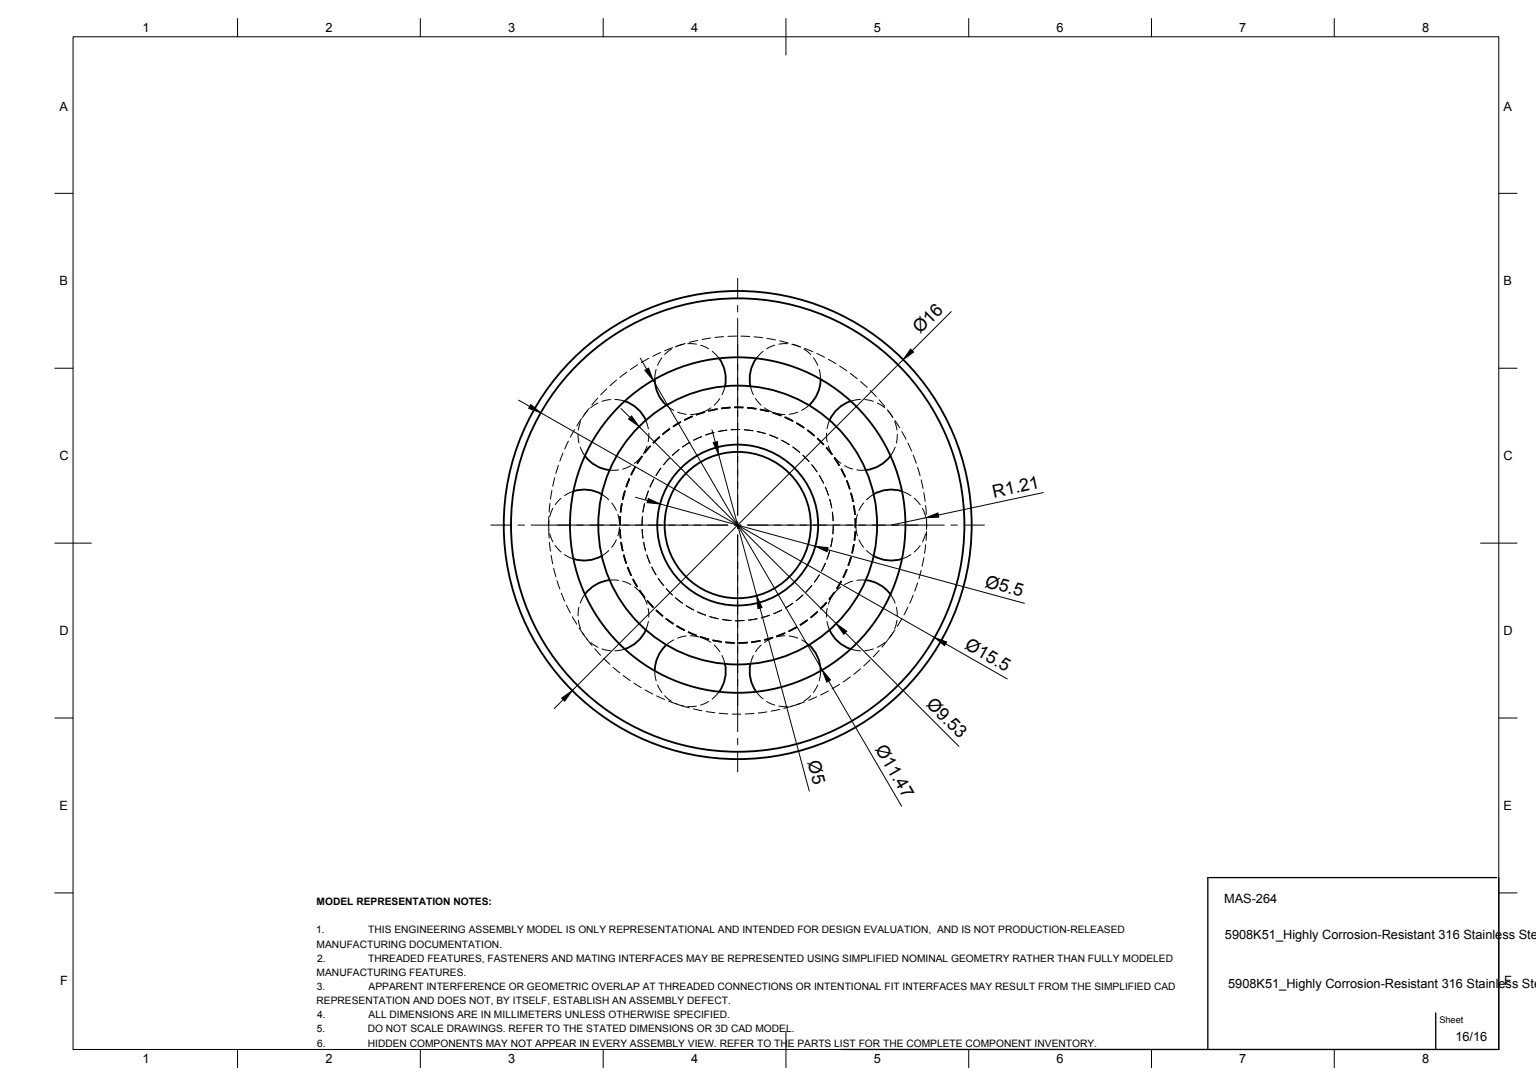
ISO-10303-21;
HEADER;
/* Generated by software containing ST-Developer
 * from STEP Tools, Inc. (www.steptools.com) 
 */

FILE_DESCRIPTION(
/* description */ (''),
/* implementation_level */ '2;1');

FILE_NAME(
/* name */ '5908K51_Highly Corrosion-Resistant 316 Stainless Steel Ball Bearing.step',
/* time_stamp */ '2026-10-12T15:37:13-07:00',
/* author */ (''),
/* organization */ (''),
/* preprocessor_version */ 'ST-DEVELOPER v20.2',
/* originating_system */ 'Autodesk Translation Framework v15.15.0.0',
/* authorisation */ '');

FILE_SCHEMA (('AUTOMOTIVE_DESIGN { 1 0 10303 214 3 1 1 }'));
ENDSEC;

DATA;
#10=MECHANICAL_DESIGN_GEOMETRIC_PRESENTATION_REPRESENTATION('',(#337,#338,#339,#340,#341,#342,#343,#344,#345,#346,#347,#348,#349),#36460);
#95=SPHERICAL_SURFACE('',#11984,1.21175743903915);
#96=SPHERICAL_SURFACE('',#11986,1.21175743903915);
#97=SPHERICAL_SURFACE('',#11988,1.21175743903915);
#98=SPHERICAL_SURFACE('',#11990,1.21175743903915);
#99=SPHERICAL_SURFACE('',#11992,1.21175743903915);
#100=SPHERICAL_SURFACE('',#11994,1.21175743903915);
#101=SPHERICAL_SURFACE('',#11996,1.21175743903915);
#102=SPHERICAL_SURFACE('',#11998,1.21175743903915);
#103=SPHERICAL_SURFACE('',#12000,1.21175743903915);
#104=SPHERICAL_SURFACE('',#12002,1.21175743903915);
#110=SHAPE_REPRESENTATION_RELATIONSHIP('SRR','None',#36522,#123);
#123=ADVANCED_BREP_SHAPE_REPRESENTATION('',(#369,#370,#371,#372,#373,#374,
#375,#376,#377,#378,#379,#380,#381),#36451);
#165=FACE_BOUND('',#2009,.T.);
#166=FACE_BOUND('',#2011,.T.);
#167=FACE_BOUND('',#2017,.T.);
#168=FACE_BOUND('',#2019,.T.);
#169=FACE_BOUND('',#2028,.T.);
#170=FACE_BOUND('',#2030,.T.);
#171=FACE_BOUND('',#2032,.T.);
#319=CONICAL_SURFACE('',#11939,7.75,0.785398163397447);
#320=CONICAL_SURFACE('',#11945,8.,0.785398163397448);
#321=CONICAL_SURFACE('',#11958,4.01780239848197,0.78539816339745);
#322=CONICAL_SURFACE('',#11962,3.26912128048043,0.78539816339745);
#323=CONICAL_SURFACE('',#11968,2.5,0.785398163397447);
#324=CONICAL_SURFACE('',#11979,3.26912128048043,0.78539816339745);
#337=STYLED_ITEM('',(#36596),#369);
#338=STYLED_ITEM('',(#36596),#370);
#339=STYLED_ITEM('',(#36596),#371);
#340=STYLED_ITEM('',(#36596),#372);
#341=STYLED_ITEM('',(#36596),#373);
#342=STYLED_ITEM('',(#36596),#374);
#343=STYLED_ITEM('',(#36596),#375);
#344=STYLED_ITEM('',(#36596),#376);
#345=STYLED_ITEM('',(#36596),#377);
#346=STYLED_ITEM('',(#36596),#378);
#347=STYLED_ITEM('',(#36596),#379);
#348=STYLED_ITEM('',(#36596),#380);
#349=STYLED_ITEM('',(#36596),#381);
#369=MANIFOLD_SOLID_BREP('Body1',#11273);
#370=MANIFOLD_SOLID_BREP('Body2',#11274);
#371=MANIFOLD_SOLID_BREP('Body3',#11275);
#372=MANIFOLD_SOLID_BREP('Body4',#11276);
#373=MANIFOLD_SOLID_BREP('Body5',#11277);
#374=MANIFOLD_SOLID_BREP('Body6',#11278);
#375=MANIFOLD_SOLID_BREP('Body7',#11279);
#376=MANIFOLD_SOLID_BREP('Body8',#11280);
#377=MANIFOLD_SOLID_BREP('Body9',#11281);
#378=MANIFOLD_SOLID_BREP('Body10',#11282);
#379=MANIFOLD_SOLID_BREP('Body11',#11283);
#380=MANIFOLD_SOLID_BREP('Body12',#11284);
#381=MANIFOLD_SOLID_BREP('Body13',#11285);
#533=PLANE('',#11947);
#534=PLANE('',#11948);
#535=PLANE('',#11960);
#536=PLANE('',#11961);
#537=PLANE('',#11981);
#538=PLANE('',#11982);
#539=PLANE('',#11983);
#1023=TOROIDAL_SURFACE('',#11934,5.25,1.21175743903915);
#1024=TOROIDAL_SURFACE('',#11952,5.25,1.21175743903915);
#1025=TOROIDAL_SURFACE('',#11973,5.25,1.21175743903915);
#1355=FACE_OUTER_BOUND('',#2002,.T.);
#1356=FACE_OUTER_BOUND('',#2003,.T.);
#1357=FACE_OUTER_BOUND('',#2004,.T.);
#1358=FACE_OUTER_BOUND('',#2005,.T.);
#1359=FACE_OUTER_BOUND('',#2006,.T.);
#1360=FACE_OUTER_BOUND('',#2007,.T.);
#1361=FACE_OUTER_BOUND('',#2008,.T.);
#1362=FACE_OUTER_BOUND('',#2010,.T.);
#1363=FACE_OUTER_BOUND('',#2012,.T.);
#1364=FACE_OUTER_BOUND('',#2013,.T.);
#1365=FACE_OUTER_BOUND('',#2014,.T.);
#1366=FACE_OUTER_BOUND('',#2015,.T.);
#1367=FACE_OUTER_BOUND('',#2016,.T.);
#1368=FACE_OUTER_BOUND('',#2018,.T.);
#1369=FACE_OUTER_BOUND('',#2020,.T.);
#1370=FACE_OUTER_BOUND('',#2021,.T.);
#1371=FACE_OUTER_BOUND('',#2022,.T.);
#1372=FACE_OUTER_BOUND('',#2023,.T.);
#1373=FACE_OUTER_BOUND('',#2024,.T.);
#1374=FACE_OUTER_BOUND('',#2025,.T.);
#1375=FACE_OUTER_BOUND('',#2026,.T.);
#1376=FACE_OUTER_BOUND('',#2027,.T.);
#1377=FACE_OUTER_BOUND('',#2029,.T.);
#1378=FACE_OUTER_BOUND('',#2031,.T.);
#1379=FACE_OUTER_BOUND('',#2033,.T.);
#1380=FACE_OUTER_BOUND('',#2034,.T.);
#1381=FACE_OUTER_BOUND('',#2035,.T.);
#1382=FACE_OUTER_BOUND('',#2036,.T.);
#1383=FACE_OUTER_BOUND('',#2037,.T.);
#1384=FACE_OUTER_BOUND('',#2038,.T.);
#1385=FACE_OUTER_BOUND('',#2039,.T.);
#1386=FACE_OUTER_BOUND('',#2040,.T.);
#1387=FACE_OUTER_BOUND('',#2041,.T.);
#1388=FACE_OUTER_BOUND('',#2042,.T.);
#2002=EDGE_LOOP('',(#8944,#8945,#8946,#8947));
#2003=EDGE_LOOP('',(#8948,#8949,#8950,#8951));
#2004=EDGE_LOOP('',(#8952,#8953,#8954,#8955));
#2005=EDGE_LOOP('',(#8956,#8957,#8958,#8959));
#2006=EDGE_LOOP('',(#8960,#8961,#8962,#8963,#8964));
#2007=EDGE_LOOP('',(#8965,#8966,#8967,#8968,#8969));
#2008=EDGE_LOOP('',(#8970));
#2009=EDGE_LOOP('',(#8971));
#2010=EDGE_LOOP('',(#8972));
#2011=EDGE_LOOP('',(#8973));
#2012=EDGE_LOOP('',(#8974,#8975,#8976,#8977));
#2013=EDGE_LOOP('',(#8978,#8979,#8980,#8981));
#2014=EDGE_LOOP('',(#8982,#8983,#8984,#8985));
#2015=EDGE_LOOP('',(#8986,#8987,#8988,#8989));
#2016=EDGE_LOOP('',(#8990));
#2017=EDGE_LOOP('',(#8991));
#2018=EDGE_LOOP('',(#8992));
#2019=EDGE_LOOP('',(#8993));
#2020=EDGE_LOOP('',(#8994,#8995,#8996,#8997));
#2021=EDGE_LOOP('',(#8998,#8999,#9000,#9001,#9002));
#2022=EDGE_LOOP('',(#9003,#9004,#9005,#9006,#9007));
#2023=EDGE_LOOP('',(#9008,#9009,#9010,#9011));
#2024=EDGE_LOOP('',(#9012,#9013,#9014,#9015));
#2025=EDGE_LOOP('',(#9016,#9017,#9018,#9019));
#2026=EDGE_LOOP('',(#9020,#9021,#9022,#9023));
#2027=EDGE_LOOP('',(#9024));
#2028=EDGE_LOOP('',(#9025));
#2029=EDGE_LOOP('',(#9026));
#2030=EDGE_LOOP('',(#9027));
#2031=EDGE_LOOP('',(#9028));
#2032=EDGE_LOOP('',(#9029));
#2033=EDGE_LOOP('',(#9030,#9031));
#2034=EDGE_LOOP('',(#9032,#9033));
#2035=EDGE_LOOP('',(#9034,#9035));
#2036=EDGE_LOOP('',(#9036,#9037));
#2037=EDGE_LOOP('',(#9038,#9039));
#2038=EDGE_LOOP('',(#9040,#9041));
#2039=EDGE_LOOP('',(#9042,#9043));
#2040=EDGE_LOOP('',(#9044,#9045));
#2041=EDGE_LOOP('',(#9046,#9047));
#2042=EDGE_LOOP('',(#9048,#9049));
#2798=LINE('',#34750,#3744);
#2799=LINE('',#34759,#3745);
#2800=LINE('',#34764,#3746);
#2801=LINE('',#34771,#3747);
#2802=LINE('',#34774,#3748);
#2803=LINE('',#34782,#3749);
#2804=LINE('',#34792,#3750);
#2805=LINE('',#34796,#3751);
#2806=LINE('',#34804,#3752);
#2807=LINE('',#34811,#3753);
#2808=LINE('',#34814,#3754);
#2809=LINE('',#34820,#3755);
#2810=LINE('',#34830,#3756);
#2811=LINE('',#34835,#3757);
#3744=VECTOR('',#13837,5.73351648351648);
#3745=VECTOR('',#13850,5.73351648351648);
#3746=VECTOR('',#13855,7.75);
#3747=VECTOR('',#13864,8.);
#3748=VECTOR('',#13867,8.);
#3749=VECTOR('',#13878,4.76648351648352);
#3750=VECTOR('',#13891,3.26912128048043);
#3751=VECTOR('',#13896,4.01780239848197);
#3752=VECTOR('',#13907,3.26912128048043);
#3753=VECTOR('',#13916,2.5);
#3754=VECTOR('',#13919,2.5);
#3755=VECTOR('',#13926,4.76648351648352);
#3756=VECTOR('',#13939,3.26912128048043);
#3757=VECTOR('',#13946,3.26912128048043);
#4402=CIRCLE('',#11932,5.73351648351648);
#4403=CIRCLE('',#11933,5.73351648351648);
#4404=CIRCLE('',#11935,5.73351648351648);
#4405=CIRCLE('',#11936,1.21175743903915);
#4406=CIRCLE('',#11938,5.73351648351648);
#4407=CIRCLE('',#11940,8.);
#4408=CIRCLE('',#11941,7.75);
#4409=CIRCLE('',#11943,8.);
#4410=CIRCLE('',#11944,8.);
#4411=CIRCLE('',#11946,7.75);
#4412=CIRCLE('',#11950,4.76648351648352);
#4413=CIRCLE('',#11951,4.76648351648352);
#4414=CIRCLE('',#11953,1.21175743903915);
#4415=CIRCLE('',#11954,4.03824256096085);
#4416=CIRCLE('',#11956,3.26912128048043);
#4417=CIRCLE('',#11957,3.26912128048043);
#4418=CIRCLE('',#11959,4.01780239848197);
#4419=CIRCLE('',#11963,2.5);
#4420=CIRCLE('',#11964,3.26912128048043);
#4421=CIRCLE('',#11966,2.5);
#4422=CIRCLE('',#11967,2.5);
#4423=CIRCLE('',#11969,2.75);
#4424=CIRCLE('',#11971,4.76648351648352);
#4425=CIRCLE('',#11972,4.76648351648352);
#4426=CIRCLE('',#11974,4.03824256096085);
#4427=CIRCLE('',#11975,1.21175743903915);
#4428=CIRCLE('',#11977,3.26912128048043);
#4429=CIRCLE('',#11978,3.26912128048043);
#4430=CIRCLE('',#11980,4.01780239848197);
#4431=CIRCLE('',#11985,1.21175743903915);
#4432=CIRCLE('',#11987,1.21175743903915);
#4433=CIRCLE('',#11989,1.21175743903915);
#4434=CIRCLE('',#11991,1.21175743903915);
#4435=CIRCLE('',#11993,1.21175743903915);
#4436=CIRCLE('',#11995,1.21175743903915);
#4437=CIRCLE('',#11997,1.21175743903915);
#4438=CIRCLE('',#11999,1.21175743903915);
#4439=CIRCLE('',#12001,1.21175743903915);
#4440=CIRCLE('',#12003,1.21175743903915);
#5153=VERTEX_POINT('',#34747);
#5154=VERTEX_POINT('',#34749);
#5155=VERTEX_POINT('',#34753);
#5156=VERTEX_POINT('',#34757);
#5157=VERTEX_POINT('',#34761);
#5158=VERTEX_POINT('',#34763);
#5159=VERTEX_POINT('',#34767);
#5160=VERTEX_POINT('',#34768);
#5161=VERTEX_POINT('',#34773);
#5162=VERTEX_POINT('',#34779);
#5163=VERTEX_POINT('',#34781);
#5164=VERTEX_POINT('',#34785);
#5165=VERTEX_POINT('',#34789);
#5166=VERTEX_POINT('',#34791);
#5167=VERTEX_POINT('',#34795);
#5168=VERTEX_POINT('',#34801);
#5169=VERTEX_POINT('',#34803);
#5170=VERTEX_POINT('',#34807);
#5171=VERTEX_POINT('',#34808);
#5172=VERTEX_POINT('',#34813);
#5173=VERTEX_POINT('',#34817);
#5174=VERTEX_POINT('',#34819);
#5175=VERTEX_POINT('',#34823);
#5176=VERTEX_POINT('',#34827);
#5177=VERTEX_POINT('',#34829);
#5178=VERTEX_POINT('',#34833);
#5179=VERTEX_POINT('',#34840);
#5180=VERTEX_POINT('',#34841);
#5181=VERTEX_POINT('',#34844);
#5182=VERTEX_POINT('',#34845);
#5183=VERTEX_POINT('',#34848);
#5184=VERTEX_POINT('',#34849);
#5185=VERTEX_POINT('',#34852);
#5186=VERTEX_POINT('',#34853);
#5187=VERTEX_POINT('',#34856);
#5188=VERTEX_POINT('',#34857);
#5189=VERTEX_POINT('',#34860);
#5190=VERTEX_POINT('',#34861);
#5191=VERTEX_POINT('',#34864);
#5192=VERTEX_POINT('',#34865);
#5193=VERTEX_POINT('',#34868);
#5194=VERTEX_POINT('',#34869);
#5195=VERTEX_POINT('',#34872);
#5196=VERTEX_POINT('',#34873);
#5197=VERTEX_POINT('',#34876);
#5198=VERTEX_POINT('',#34877);
#6503=EDGE_CURVE('',#5153,#5153,#4402,.T.);
#6504=EDGE_CURVE('',#5153,#5154,#2798,.T.);
#6505=EDGE_CURVE('',#5154,#5154,#4403,.T.);
#6506=EDGE_CURVE('',#5155,#5155,#4404,.T.);
#6507=EDGE_CURVE('',#5155,#5153,#4405,.T.);
#6508=EDGE_CURVE('',#5156,#5156,#4406,.T.);
#6509=EDGE_CURVE('',#5156,#5155,#2799,.T.);
#6510=EDGE_CURVE('',#5157,#5157,#4407,.T.);
#6511=EDGE_CURVE('',#5157,#5158,#2800,.T.);
#6512=EDGE_CURVE('',#5158,#5158,#4408,.T.);
#6513=EDGE_CURVE('',#5159,#5160,#4409,.T.);
#6514=EDGE_CURVE('',#5160,#5159,#4410,.T.);
#6515=EDGE_CURVE('',#5160,#5157,#2801,.T.);
#6516=EDGE_CURVE('',#5159,#5161,#2802,.T.);
#6517=EDGE_CURVE('',#5161,#5161,#4411,.T.);
#6518=EDGE_CURVE('',#5162,#5162,#4412,.T.);
#6519=EDGE_CURVE('',#5162,#5163,#2803,.T.);
#6520=EDGE_CURVE('',#5163,#5163,#4413,.T.);
#6521=EDGE_CURVE('',#5163,#5164,#4414,.T.);
#6522=EDGE_CURVE('',#5164,#5164,#4415,.T.);
#6523=EDGE_CURVE('',#5165,#5165,#4416,.T.);
#6524=EDGE_CURVE('',#5165,#5166,#2804,.T.);
#6525=EDGE_CURVE('',#5166,#5166,#4417,.T.);
#6526=EDGE_CURVE('',#5166,#5167,#2805,.T.);
#6527=EDGE_CURVE('',#5167,#5167,#4418,.T.);
#6528=EDGE_CURVE('',#5168,#5168,#4419,.T.);
#6529=EDGE_CURVE('',#5168,#5169,#2806,.T.);
#6530=EDGE_CURVE('',#5169,#5169,#4420,.T.);
#6531=EDGE_CURVE('',#5170,#5171,#4421,.T.);
#6532=EDGE_CURVE('',#5171,#5170,#4422,.T.);
#6533=EDGE_CURVE('',#5171,#5168,#2807,.T.);
#6534=EDGE_CURVE('',#5170,#5172,#2808,.T.);
#6535=EDGE_CURVE('',#5172,#5172,#4423,.T.);
#6536=EDGE_CURVE('',#5173,#5173,#4424,.T.);
#6537=EDGE_CURVE('',#5173,#5174,#2809,.T.);
#6538=EDGE_CURVE('',#5174,#5174,#4425,.T.);
#6539=EDGE_CURVE('',#5175,#5175,#4426,.T.);
#6540=EDGE_CURVE('',#5175,#5173,#4427,.T.);
#6541=EDGE_CURVE('',#5176,#5176,#4428,.T.);
#6542=EDGE_CURVE('',#5176,#5177,#2810,.T.);
#6543=EDGE_CURVE('',#5177,#5177,#4429,.T.);
#6544=EDGE_CURVE('',#5178,#5178,#4430,.T.);
#6545=EDGE_CURVE('',#5178,#5176,#2811,.T.);
#6546=EDGE_CURVE('',#5179,#5180,#4431,.T.);
#6547=EDGE_CURVE('',#5181,#5182,#4432,.T.);
#6548=EDGE_CURVE('',#5183,#5184,#4433,.T.);
#6549=EDGE_CURVE('',#5185,#5186,#4434,.T.);
#6550=EDGE_CURVE('',#5187,#5188,#4435,.T.);
#6551=EDGE_CURVE('',#5189,#5190,#4436,.T.);
#6552=EDGE_CURVE('',#5191,#5192,#4437,.T.);
#6553=EDGE_CURVE('',#5193,#5194,#4438,.T.);
#6554=EDGE_CURVE('',#5195,#5196,#4439,.T.);
#6555=EDGE_CURVE('',#5197,#5198,#4440,.T.);
#8944=ORIENTED_EDGE('',*,*,#6503,.F.);
#8945=ORIENTED_EDGE('',*,*,#6504,.T.);
#8946=ORIENTED_EDGE('',*,*,#6505,.T.);
#8947=ORIENTED_EDGE('',*,*,#6504,.F.);
#8948=ORIENTED_EDGE('',*,*,#6506,.F.);
#8949=ORIENTED_EDGE('',*,*,#6507,.T.);
#8950=ORIENTED_EDGE('',*,*,#6503,.T.);
#8951=ORIENTED_EDGE('',*,*,#6507,.F.);
#8952=ORIENTED_EDGE('',*,*,#6508,.F.);
#8953=ORIENTED_EDGE('',*,*,#6509,.T.);
#8954=ORIENTED_EDGE('',*,*,#6506,.T.);
#8955=ORIENTED_EDGE('',*,*,#6509,.F.);
#8956=ORIENTED_EDGE('',*,*,#6510,.F.);
#8957=ORIENTED_EDGE('',*,*,#6511,.T.);
#8958=ORIENTED_EDGE('',*,*,#6512,.T.);
#8959=ORIENTED_EDGE('',*,*,#6511,.F.);
#8960=ORIENTED_EDGE('',*,*,#6513,.F.);
#8961=ORIENTED_EDGE('',*,*,#6514,.F.);
#8962=ORIENTED_EDGE('',*,*,#6515,.T.);
#8963=ORIENTED_EDGE('',*,*,#6510,.T.);
#8964=ORIENTED_EDGE('',*,*,#6515,.F.);
#8965=ORIENTED_EDGE('',*,*,#6513,.T.);
#8966=ORIENTED_EDGE('',*,*,#6514,.T.);
#8967=ORIENTED_EDGE('',*,*,#6516,.T.);
#8968=ORIENTED_EDGE('',*,*,#6517,.F.);
#8969=ORIENTED_EDGE('',*,*,#6516,.F.);
#8970=ORIENTED_EDGE('',*,*,#6512,.F.);
#8971=ORIENTED_EDGE('',*,*,#6508,.T.);
#8972=ORIENTED_EDGE('',*,*,#6517,.T.);
#8973=ORIENTED_EDGE('',*,*,#6505,.F.);
#8974=ORIENTED_EDGE('',*,*,#6518,.F.);
#8975=ORIENTED_EDGE('',*,*,#6519,.T.);
#8976=ORIENTED_EDGE('',*,*,#6520,.T.);
#8977=ORIENTED_EDGE('',*,*,#6519,.F.);
#8978=ORIENTED_EDGE('',*,*,#6520,.F.);
#8979=ORIENTED_EDGE('',*,*,#6521,.T.);
#8980=ORIENTED_EDGE('',*,*,#6522,.T.);
#8981=ORIENTED_EDGE('',*,*,#6521,.F.);
#8982=ORIENTED_EDGE('',*,*,#6523,.F.);
#8983=ORIENTED_EDGE('',*,*,#6524,.T.);
#8984=ORIENTED_EDGE('',*,*,#6525,.T.);
#8985=ORIENTED_EDGE('',*,*,#6524,.F.);
#8986=ORIENTED_EDGE('',*,*,#6525,.F.);
#8987=ORIENTED_EDGE('',*,*,#6526,.T.);
#8988=ORIENTED_EDGE('',*,*,#6527,.T.);
#8989=ORIENTED_EDGE('',*,*,#6526,.F.);
#8990=ORIENTED_EDGE('',*,*,#6518,.T.);
#8991=ORIENTED_EDGE('',*,*,#6527,.F.);
#8992=ORIENTED_EDGE('',*,*,#6522,.F.);
#8993=ORIENTED_EDGE('',*,*,#6523,.T.);
#8994=ORIENTED_EDGE('',*,*,#6528,.F.);
#8995=ORIENTED_EDGE('',*,*,#6529,.T.);
#8996=ORIENTED_EDGE('',*,*,#6530,.T.);
#8997=ORIENTED_EDGE('',*,*,#6529,.F.);
#8998=ORIENTED_EDGE('',*,*,#6531,.F.);
#8999=ORIENTED_EDGE('',*,*,#6532,.F.);
#9000=ORIENTED_EDGE('',*,*,#6533,.T.);
#9001=ORIENTED_EDGE('',*,*,#6528,.T.);
#9002=ORIENTED_EDGE('',*,*,#6533,.F.);
#9003=ORIENTED_EDGE('',*,*,#6531,.T.);
#9004=ORIENTED_EDGE('',*,*,#6532,.T.);
#9005=ORIENTED_EDGE('',*,*,#6534,.T.);
#9006=ORIENTED_EDGE('',*,*,#6535,.F.);
#9007=ORIENTED_EDGE('',*,*,#6534,.F.);
#9008=ORIENTED_EDGE('',*,*,#6536,.F.);
#9009=ORIENTED_EDGE('',*,*,#6537,.T.);
#9010=ORIENTED_EDGE('',*,*,#6538,.T.);
#9011=ORIENTED_EDGE('',*,*,#6537,.F.);
#9012=ORIENTED_EDGE('',*,*,#6539,.F.);
#9013=ORIENTED_EDGE('',*,*,#6540,.T.);
#9014=ORIENTED_EDGE('',*,*,#6536,.T.);
#9015=ORIENTED_EDGE('',*,*,#6540,.F.);
#9016=ORIENTED_EDGE('',*,*,#6541,.F.);
#9017=ORIENTED_EDGE('',*,*,#6542,.T.);
#9018=ORIENTED_EDGE('',*,*,#6543,.T.);
#9019=ORIENTED_EDGE('',*,*,#6542,.F.);
#9020=ORIENTED_EDGE('',*,*,#6544,.F.);
#9021=ORIENTED_EDGE('',*,*,#6545,.T.);
#9022=ORIENTED_EDGE('',*,*,#6541,.T.);
#9023=ORIENTED_EDGE('',*,*,#6545,.F.);
#9024=ORIENTED_EDGE('',*,*,#6544,.T.);
#9025=ORIENTED_EDGE('',*,*,#6530,.F.);
#9026=ORIENTED_EDGE('',*,*,#6539,.T.);
#9027=ORIENTED_EDGE('',*,*,#6543,.F.);
#9028=ORIENTED_EDGE('',*,*,#6538,.F.);
#9029=ORIENTED_EDGE('',*,*,#6535,.T.);
#9030=ORIENTED_EDGE('',*,*,#6546,.T.);
#9031=ORIENTED_EDGE('',*,*,#6546,.F.);
#9032=ORIENTED_EDGE('',*,*,#6547,.T.);
#9033=ORIENTED_EDGE('',*,*,#6547,.F.);
#9034=ORIENTED_EDGE('',*,*,#6548,.T.);
#9035=ORIENTED_EDGE('',*,*,#6548,.F.);
#9036=ORIENTED_EDGE('',*,*,#6549,.T.);
#9037=ORIENTED_EDGE('',*,*,#6549,.F.);
#9038=ORIENTED_EDGE('',*,*,#6550,.T.);
#9039=ORIENTED_EDGE('',*,*,#6550,.F.);
#9040=ORIENTED_EDGE('',*,*,#6551,.T.);
#9041=ORIENTED_EDGE('',*,*,#6551,.F.);
#9042=ORIENTED_EDGE('',*,*,#6552,.T.);
#9043=ORIENTED_EDGE('',*,*,#6552,.F.);
#9044=ORIENTED_EDGE('',*,*,#6553,.T.);
#9045=ORIENTED_EDGE('',*,*,#6553,.F.);
#9046=ORIENTED_EDGE('',*,*,#6554,.T.);
#9047=ORIENTED_EDGE('',*,*,#6554,.F.);
#9048=ORIENTED_EDGE('',*,*,#6555,.T.);
#9049=ORIENTED_EDGE('',*,*,#6555,.F.);
#10565=CYLINDRICAL_SURFACE('',#11931,5.73351648351648);
#10566=CYLINDRICAL_SURFACE('',#11937,5.73351648351648);
#10567=CYLINDRICAL_SURFACE('',#11942,8.);
#10568=CYLINDRICAL_SURFACE('',#11949,4.76648351648352);
#10569=CYLINDRICAL_SURFACE('',#11955,3.26912128048043);
#10570=CYLINDRICAL_SURFACE('',#11965,2.5);
#10571=CYLINDRICAL_SURFACE('',#11970,4.76648351648352);
#10572=CYLINDRICAL_SURFACE('',#11976,3.26912128048043);
#10976=ADVANCED_FACE('',(#1355),#10565,.F.);
#10977=ADVANCED_FACE('',(#1356),#1023,.F.);
#10978=ADVANCED_FACE('',(#1357),#10566,.F.);
#10979=ADVANCED_FACE('',(#1358),#319,.T.);
#10980=ADVANCED_FACE('',(#1359),#10567,.T.);
#10981=ADVANCED_FACE('',(#1360),#320,.T.);
#10982=ADVANCED_FACE('',(#1361,#165),#533,.F.);
#10983=ADVANCED_FACE('',(#1362,#166),#534,.F.);
#10984=ADVANCED_FACE('',(#1363),#10568,.T.);
#10985=ADVANCED_FACE('',(#1364),#1024,.F.);
#10986=ADVANCED_FACE('',(#1365),#10569,.F.);
#10987=ADVANCED_FACE('',(#1366),#321,.F.);
#10988=ADVANCED_FACE('',(#1367,#167),#535,.F.);
#10989=ADVANCED_FACE('',(#1368,#168),#536,.F.);
#10990=ADVANCED_FACE('',(#1369),#322,.F.);
#10991=ADVANCED_FACE('',(#1370),#10570,.F.);
#10992=ADVANCED_FACE('',(#1371),#323,.F.);
#10993=ADVANCED_FACE('',(#1372),#10571,.T.);
#10994=ADVANCED_FACE('',(#1373),#1025,.F.);
#10995=ADVANCED_FACE('',(#1374),#10572,.T.);
#10996=ADVANCED_FACE('',(#1375),#324,.T.);
#10997=ADVANCED_FACE('',(#1376,#169),#537,.F.);
#10998=ADVANCED_FACE('',(#1377,#170),#538,.F.);
#10999=ADVANCED_FACE('',(#1378,#171),#539,.F.);
#11000=ADVANCED_FACE('',(#1379),#95,.T.);
#11001=ADVANCED_FACE('',(#1380),#96,.T.);
#11002=ADVANCED_FACE('',(#1381),#97,.T.);
#11003=ADVANCED_FACE('',(#1382),#98,.T.);
#11004=ADVANCED_FACE('',(#1383),#99,.T.);
#11005=ADVANCED_FACE('',(#1384),#100,.T.);
#11006=ADVANCED_FACE('',(#1385),#101,.T.);
#11007=ADVANCED_FACE('',(#1386),#102,.T.);
#11008=ADVANCED_FACE('',(#1387),#103,.T.);
#11009=ADVANCED_FACE('',(#1388),#104,.T.);
#11273=CLOSED_SHELL('',(#10976,#10977,#10978,#10979,#10980,#10981,#10982,
#10983));
#11274=CLOSED_SHELL('',(#10984,#10985,#10986,#10987,#10988,#10989));
#11275=CLOSED_SHELL('',(#10990,#10991,#10992,#10993,#10994,#10995,#10996,
#10997,#10998,#10999));
#11276=CLOSED_SHELL('',(#11000));
#11277=CLOSED_SHELL('',(#11001));
#11278=CLOSED_SHELL('',(#11002));
#11279=CLOSED_SHELL('',(#11003));
#11280=CLOSED_SHELL('',(#11004));
#11281=CLOSED_SHELL('',(#11005));
#11282=CLOSED_SHELL('',(#11006));
#11283=CLOSED_SHELL('',(#11007));
#11284=CLOSED_SHELL('',(#11008));
#11285=CLOSED_SHELL('',(#11009));
#11930=AXIS2_PLACEMENT_3D('',#34745,#13831,#13832);
#11931=AXIS2_PLACEMENT_3D('',#34746,#13833,#13834);
#11932=AXIS2_PLACEMENT_3D('',#34748,#13835,#13836);
#11933=AXIS2_PLACEMENT_3D('',#34751,#13838,#13839);
#11934=AXIS2_PLACEMENT_3D('',#34752,#13840,#13841);
#11935=AXIS2_PLACEMENT_3D('',#34754,#13842,#13843);
#11936=AXIS2_PLACEMENT_3D('',#34755,#13844,#13845);
#11937=AXIS2_PLACEMENT_3D('',#34756,#13846,#13847);
#11938=AXIS2_PLACEMENT_3D('',#34758,#13848,#13849);
#11939=AXIS2_PLACEMENT_3D('',#34760,#13851,#13852);
#11940=AXIS2_PLACEMENT_3D('',#34762,#13853,#13854);
#11941=AXIS2_PLACEMENT_3D('',#34765,#13856,#13857);
#11942=AXIS2_PLACEMENT_3D('',#34766,#13858,#13859);
#11943=AXIS2_PLACEMENT_3D('',#34769,#13860,#13861);
#11944=AXIS2_PLACEMENT_3D('',#34770,#13862,#13863);
#11945=AXIS2_PLACEMENT_3D('',#34772,#13865,#13866);
#11946=AXIS2_PLACEMENT_3D('',#34775,#13868,#13869);
#11947=AXIS2_PLACEMENT_3D('',#34776,#13870,#13871);
#11948=AXIS2_PLACEMENT_3D('',#34777,#13872,#13873);
#11949=AXIS2_PLACEMENT_3D('',#34778,#13874,#13875);
#11950=AXIS2_PLACEMENT_3D('',#34780,#13876,#13877);
#11951=AXIS2_PLACEMENT_3D('',#34783,#13879,#13880);
#11952=AXIS2_PLACEMENT_3D('',#34784,#13881,#13882);
#11953=AXIS2_PLACEMENT_3D('',#34786,#13883,#13884);
#11954=AXIS2_PLACEMENT_3D('',#34787,#13885,#13886);
#11955=AXIS2_PLACEMENT_3D('',#34788,#13887,#13888);
#11956=AXIS2_PLACEMENT_3D('',#34790,#13889,#13890);
#11957=AXIS2_PLACEMENT_3D('',#34793,#13892,#13893);
#11958=AXIS2_PLACEMENT_3D('',#34794,#13894,#13895);
#11959=AXIS2_PLACEMENT_3D('',#34797,#13897,#13898);
#11960=AXIS2_PLACEMENT_3D('',#34798,#13899,#13900);
#11961=AXIS2_PLACEMENT_3D('',#34799,#13901,#13902);
#11962=AXIS2_PLACEMENT_3D('',#34800,#13903,#13904);
#11963=AXIS2_PLACEMENT_3D('',#34802,#13905,#13906);
#11964=AXIS2_PLACEMENT_3D('',#34805,#13908,#13909);
#11965=AXIS2_PLACEMENT_3D('',#34806,#13910,#13911);
#11966=AXIS2_PLACEMENT_3D('',#34809,#13912,#13913);
#11967=AXIS2_PLACEMENT_3D('',#34810,#13914,#13915);
#11968=AXIS2_PLACEMENT_3D('',#34812,#13917,#13918);
#11969=AXIS2_PLACEMENT_3D('',#34815,#13920,#13921);
#11970=AXIS2_PLACEMENT_3D('',#34816,#13922,#13923);
#11971=AXIS2_PLACEMENT_3D('',#34818,#13924,#13925);
#11972=AXIS2_PLACEMENT_3D('',#34821,#13927,#13928);
#11973=AXIS2_PLACEMENT_3D('',#34822,#13929,#13930);
#11974=AXIS2_PLACEMENT_3D('',#34824,#13931,#13932);
#11975=AXIS2_PLACEMENT_3D('',#34825,#13933,#13934);
#11976=AXIS2_PLACEMENT_3D('',#34826,#13935,#13936);
#11977=AXIS2_PLACEMENT_3D('',#34828,#13937,#13938);
#11978=AXIS2_PLACEMENT_3D('',#34831,#13940,#13941);
#11979=AXIS2_PLACEMENT_3D('',#34832,#13942,#13943);
#11980=AXIS2_PLACEMENT_3D('',#34834,#13944,#13945);
#11981=AXIS2_PLACEMENT_3D('',#34836,#13947,#13948);
#11982=AXIS2_PLACEMENT_3D('',#34837,#13949,#13950);
#11983=AXIS2_PLACEMENT_3D('',#34838,#13951,#13952);
#11984=AXIS2_PLACEMENT_3D('',#34839,#13953,#13954);
#11985=AXIS2_PLACEMENT_3D('',#34842,#13955,#13956);
#11986=AXIS2_PLACEMENT_3D('',#34843,#13957,#13958);
#11987=AXIS2_PLACEMENT_3D('',#34846,#13959,#13960);
#11988=AXIS2_PLACEMENT_3D('',#34847,#13961,#13962);
#11989=AXIS2_PLACEMENT_3D('',#34850,#13963,#13964);
#11990=AXIS2_PLACEMENT_3D('',#34851,#13965,#13966);
#11991=AXIS2_PLACEMENT_3D('',#34854,#13967,#13968);
#11992=AXIS2_PLACEMENT_3D('',#34855,#13969,#13970);
#11993=AXIS2_PLACEMENT_3D('',#34858,#13971,#13972);
#11994=AXIS2_PLACEMENT_3D('',#34859,#13973,#13974);
#11995=AXIS2_PLACEMENT_3D('',#34862,#13975,#13976);
#11996=AXIS2_PLACEMENT_3D('',#34863,#13977,#13978);
#11997=AXIS2_PLACEMENT_3D('',#34866,#13979,#13980);
#11998=AXIS2_PLACEMENT_3D('',#34867,#13981,#13982);
#11999=AXIS2_PLACEMENT_3D('',#34870,#13983,#13984);
#12000=AXIS2_PLACEMENT_3D('',#34871,#13985,#13986);
#12001=AXIS2_PLACEMENT_3D('',#34874,#13987,#13988);
#12002=AXIS2_PLACEMENT_3D('',#34875,#13989,#13990);
#12003=AXIS2_PLACEMENT_3D('',#34878,#13991,#13992);
#13831=DIRECTION('axis',(0.,0.,1.));
#13832=DIRECTION('refdir',(1.,0.,0.));
#13833=DIRECTION('center_axis',(0.,0.,1.));
#13834=DIRECTION('ref_axis',(1.,0.,0.));
#13835=DIRECTION('center_axis',(0.,0.,1.));
#13836=DIRECTION('ref_axis',(1.,0.,0.));
#13837=DIRECTION('',(0.,0.,1.));
#13838=DIRECTION('center_axis',(0.,0.,1.));
#13839=DIRECTION('ref_axis',(1.,0.,0.));
#13840=DIRECTION('center_axis',(0.,0.,1.));
#13841=DIRECTION('ref_axis',(1.,0.,0.));
#13842=DIRECTION('center_axis',(0.,0.,1.));
#13843=DIRECTION('ref_axis',(1.,0.,0.));
#13844=DIRECTION('center_axis',(-1.22464679914735E-16,1.,0.));
#13845=DIRECTION('ref_axis',(-1.,-1.22464679914735E-16,0.));
#13846=DIRECTION('center_axis',(0.,0.,1.));
#13847=DIRECTION('ref_axis',(1.,0.,0.));
#13848=DIRECTION('center_axis',(0.,0.,1.));
#13849=DIRECTION('ref_axis',(1.,0.,0.));
#13850=DIRECTION('',(0.,0.,1.));
#13851=DIRECTION('center_axis',(0.,0.,1.));
#13852=DIRECTION('ref_axis',(1.,0.,0.));
#13853=DIRECTION('center_axis',(0.,0.,1.));
#13854=DIRECTION('ref_axis',(1.,0.,0.));
#13855=DIRECTION('',(0.707106781186547,8.65956056235492E-17,-0.707106781186548));
#13856=DIRECTION('center_axis',(0.,0.,1.));
#13857=DIRECTION('ref_axis',(1.,0.,0.));
#13858=DIRECTION('center_axis',(0.,0.,1.));
#13859=DIRECTION('ref_axis',(1.,0.,0.));
#13860=DIRECTION('center_axis',(0.,0.,1.));
#13861=DIRECTION('ref_axis',(1.,0.,0.));
#13862=DIRECTION('center_axis',(0.,0.,1.));
#13863=DIRECTION('ref_axis',(1.,0.,0.));
#13864=DIRECTION('',(0.,0.,-1.));
#13865=DIRECTION('center_axis',(0.,0.,-1.));
#13866=DIRECTION('ref_axis',(-1.,0.,0.));
#13867=DIRECTION('',(-0.707106781186547,8.65956056235493E-17,0.707106781186548));
#13868=DIRECTION('center_axis',(0.,0.,1.));
#13869=DIRECTION('ref_axis',(1.,0.,0.));
#13870=DIRECTION('center_axis',(0.,0.,1.));
#13871=DIRECTION('ref_axis',(1.,0.,0.));
#13872=DIRECTION('center_axis',(0.,0.,-1.));
#13873=DIRECTION('ref_axis',(-1.,0.,0.));
#13874=DIRECTION('center_axis',(0.,0.,1.));
#13875=DIRECTION('ref_axis',(1.,0.,0.));
#13876=DIRECTION('center_axis',(0.,0.,1.));
#13877=DIRECTION('ref_axis',(1.,0.,0.));
#13878=DIRECTION('',(0.,0.,-1.));
#13879=DIRECTION('center_axis',(0.,0.,1.));
#13880=DIRECTION('ref_axis',(1.,0.,0.));
#13881=DIRECTION('center_axis',(0.,0.,1.));
#13882=DIRECTION('ref_axis',(1.,0.,0.));
#13883=DIRECTION('center_axis',(-1.22464679914735E-16,1.,0.));
#13884=DIRECTION('ref_axis',(-1.,-1.22464679914735E-16,0.));
#13885=DIRECTION('center_axis',(0.,0.,1.));
#13886=DIRECTION('ref_axis',(1.,0.,0.));
#13887=DIRECTION('center_axis',(0.,0.,1.));
#13888=DIRECTION('ref_axis',(1.,0.,0.));
#13889=DIRECTION('center_axis',(0.,0.,1.));
#13890=DIRECTION('ref_axis',(1.,0.,0.));
#13891=DIRECTION('',(0.,0.,1.));
#13892=DIRECTION('center_axis',(0.,0.,1.));
#13893=DIRECTION('ref_axis',(1.,0.,0.));
#13894=DIRECTION('center_axis',(0.,0.,1.));
#13895=DIRECTION('ref_axis',(1.,0.,0.));
#13896=DIRECTION('',(-0.707106781186549,-8.65956056235495E-17,0.707106781186546));
#13897=DIRECTION('center_axis',(0.,0.,1.));
#13898=DIRECTION('ref_axis',(1.,0.,0.));
#13899=DIRECTION('center_axis',(0.,0.,-1.));
#13900=DIRECTION('ref_axis',(-1.,0.,0.));
#13901=DIRECTION('center_axis',(0.,0.,1.));
#13902=DIRECTION('ref_axis',(1.,0.,0.));
#13903=DIRECTION('center_axis',(0.,0.,1.));
#13904=DIRECTION('ref_axis',(1.,0.,0.));
#13905=DIRECTION('center_axis',(0.,0.,1.));
#13906=DIRECTION('ref_axis',(1.,0.,0.));
#13907=DIRECTION('',(-0.707106781186549,-8.65956056235495E-17,0.707106781186546));
#13908=DIRECTION('center_axis',(0.,0.,1.));
#13909=DIRECTION('ref_axis',(1.,0.,0.));
#13910=DIRECTION('center_axis',(0.,0.,1.));
#13911=DIRECTION('ref_axis',(1.,0.,0.));
#13912=DIRECTION('center_axis',(0.,0.,1.));
#13913=DIRECTION('ref_axis',(1.,0.,0.));
#13914=DIRECTION('center_axis',(0.,0.,1.));
#13915=DIRECTION('ref_axis',(1.,0.,0.));
#13916=DIRECTION('',(0.,0.,1.));
#13917=DIRECTION('center_axis',(0.,0.,-1.));
#13918=DIRECTION('ref_axis',(-1.,0.,0.));
#13919=DIRECTION('',(0.707106781186547,-8.65956056235492E-17,-0.707106781186548));
#13920=DIRECTION('center_axis',(0.,0.,1.));
#13921=DIRECTION('ref_axis',(1.,0.,0.));
#13922=DIRECTION('center_axis',(0.,0.,1.));
#13923=DIRECTION('ref_axis',(1.,0.,0.));
#13924=DIRECTION('center_axis',(0.,0.,1.));
#13925=DIRECTION('ref_axis',(1.,0.,0.));
#13926=DIRECTION('',(0.,0.,-1.));
#13927=DIRECTION('center_axis',(0.,0.,1.));
#13928=DIRECTION('ref_axis',(1.,0.,0.));
#13929=DIRECTION('center_axis',(0.,0.,1.));
#13930=DIRECTION('ref_axis',(1.,0.,0.));
#13931=DIRECTION('center_axis',(0.,0.,1.));
#13932=DIRECTION('ref_axis',(1.,0.,0.));
#13933=DIRECTION('center_axis',(-1.22464679914735E-16,1.,0.));
#13934=DIRECTION('ref_axis',(-1.,-1.22464679914735E-16,0.));
#13935=DIRECTION('center_axis',(0.,0.,1.));
#13936=DIRECTION('ref_axis',(1.,0.,0.));
#13937=DIRECTION('center_axis',(0.,0.,1.));
#13938=DIRECTION('ref_axis',(1.,0.,0.));
#13939=DIRECTION('',(0.,0.,-1.));
#13940=DIRECTION('center_axis',(0.,0.,1.));
#13941=DIRECTION('ref_axis',(1.,0.,0.));
#13942=DIRECTION('center_axis',(0.,0.,1.));
#13943=DIRECTION('ref_axis',(1.,0.,0.));
#13944=DIRECTION('center_axis',(0.,0.,1.));
#13945=DIRECTION('ref_axis',(1.,0.,0.));
#13946=DIRECTION('',(0.707106781186549,8.65956056235495E-17,-0.707106781186546));
#13947=DIRECTION('center_axis',(0.,0.,-1.));
#13948=DIRECTION('ref_axis',(-1.,0.,0.));
#13949=DIRECTION('center_axis',(0.,0.,-1.));
#13950=DIRECTION('ref_axis',(-1.,0.,0.));
#13951=DIRECTION('center_axis',(0.,0.,1.));
#13952=DIRECTION('ref_axis',(1.,0.,0.));
#13953=DIRECTION('center_axis',(-1.,0.,0.));
#13954=DIRECTION('ref_axis',(0.,1.,0.));
#13955=DIRECTION('center_axis',(0.,1.22464679914735E-16,1.));
#13956=DIRECTION('ref_axis',(0.,-1.,1.22464679914735E-16));
#13957=DIRECTION('center_axis',(-0.809016994374946,0.587785252292475,0.));
#13958=DIRECTION('ref_axis',(0.587785252292475,0.809016994374946,0.));
#13959=DIRECTION('center_axis',(7.19829327805999E-17,9.9076007261709E-17,
1.));
#13960=DIRECTION('ref_axis',(-0.587785252292475,-0.809016994374946,1.22464679914735E-16));
#13961=DIRECTION('center_axis',(-0.309016994374945,0.951056516295154,0.));
#13962=DIRECTION('ref_axis',(0.951056516295154,0.309016994374945,0.));
#13963=DIRECTION('center_axis',(1.16470831848909E-16,3.78436673043412E-17,
1.));
#13964=DIRECTION('ref_axis',(-0.951056516295154,-0.309016994374945,1.22464679914735E-16));
#13965=DIRECTION('center_axis',(0.309016994374952,0.951056516295152,0.));
#13966=DIRECTION('ref_axis',(0.951056516295152,-0.309016994374952,0.));
#13967=DIRECTION('center_axis',(1.16470831848909E-16,-3.78436673043421E-17,
1.));
#13968=DIRECTION('ref_axis',(-0.951056516295152,0.309016994374952,1.22464679914735E-16));
#13969=DIRECTION('center_axis',(0.809016994374951,0.587785252292469,0.));
#13970=DIRECTION('ref_axis',(0.587785252292469,-0.809016994374951,0.));
#13971=DIRECTION('center_axis',(7.19829327805991E-17,-9.90760072617096E-17,
1.));
#13972=DIRECTION('ref_axis',(-0.587785252292469,0.809016994374951,1.22464679914735E-16));
#13973=DIRECTION('center_axis',(1.,-7.32967169076673E-15,0.));
#13974=DIRECTION('ref_axis',(-7.32967169076675E-15,-1.,0.));
#13975=DIRECTION('center_axis',(-8.97625897489847E-31,-1.22464679914735E-16,
1.));
#13976=DIRECTION('ref_axis',(7.32967169076675E-15,1.,1.22464679914735E-16));
#13977=DIRECTION('center_axis',(0.809016994374942,-0.587785252292481,0.));
#13978=DIRECTION('ref_axis',(-0.587785252292481,-0.809016994374942,0.));
#13979=DIRECTION('center_axis',(-7.19829327806006E-17,-9.90760072617085E-17,
1.));
#13980=DIRECTION('ref_axis',(0.587785252292481,0.809016994374942,1.22464679914735E-16));
#13981=DIRECTION('center_axis',(0.309016994374938,-0.951056516295157,0.));
#13982=DIRECTION('ref_axis',(-0.951056516295157,-0.309016994374938,0.));
#13983=DIRECTION('center_axis',(-1.1647083184891E-16,-3.78436673043403E-17,
1.));
#13984=DIRECTION('ref_axis',(0.951056516295157,0.309016994374938,1.22464679914735E-16));
#13985=DIRECTION('center_axis',(-0.309016994374958,-0.95105651629515,0.));
#13986=DIRECTION('ref_axis',(-0.95105651629515,0.309016994374958,0.));
#13987=DIRECTION('center_axis',(-1.16470831848909E-16,3.78436673043428E-17,
1.));
#13988=DIRECTION('ref_axis',(0.95105651629515,-0.309016994374958,1.22464679914735E-16));
#13989=DIRECTION('center_axis',(-0.809016994374955,-0.587785252292462,0.));
#13990=DIRECTION('ref_axis',(-0.587785252292462,0.809016994374955,0.));
#13991=DIRECTION('center_axis',(-7.19829327805983E-17,9.90760072617101E-17,
1.));
#13992=DIRECTION('ref_axis',(0.587785252292462,-0.809016994374955,1.22464679914735E-16));
#34745=CARTESIAN_POINT('',(0.,0.,0.));
#34746=CARTESIAN_POINT('Origin',(0.,0.,2.5));
#34747=CARTESIAN_POINT('',(-5.73351648351648,-7.02153260939705E-16,1.11111111111111));
#34748=CARTESIAN_POINT('Origin',(0.,0.,1.11111111111111));
#34749=CARTESIAN_POINT('',(-5.73351648351648,-7.02153260939705E-16,2.5));
#34750=CARTESIAN_POINT('',(-5.73351648351648,-7.02153260939705E-16,2.5));
#34751=CARTESIAN_POINT('Origin',(0.,0.,2.5));
#34752=CARTESIAN_POINT('Origin',(0.,0.,-7.04171909509728E-16));
#34753=CARTESIAN_POINT('',(-5.73351648351648,-7.02153260939705E-16,-1.11111111111111));
#34754=CARTESIAN_POINT('Origin',(0.,0.,-1.11111111111111));
#34755=CARTESIAN_POINT('Origin',(-5.25,-6.42939569552361E-16,-7.04171909509728E-16));
#34756=CARTESIAN_POINT('Origin',(0.,0.,2.5));
#34757=CARTESIAN_POINT('',(-5.73351648351648,-7.02153260939705E-16,-2.5));
#34758=CARTESIAN_POINT('Origin',(0.,0.,-2.5));
#34759=CARTESIAN_POINT('',(-5.73351648351648,-7.02153260939705E-16,2.5));
#34760=CARTESIAN_POINT('Origin',(0.,0.,-2.5));
#34761=CARTESIAN_POINT('',(-8.,-9.79717439317883E-16,-2.25));
#34762=CARTESIAN_POINT('Origin',(0.,0.,-2.25));
#34763=CARTESIAN_POINT('',(-7.75,-9.49101269339199E-16,-2.5));
#34764=CARTESIAN_POINT('',(-7.75,-9.49101269339199E-16,-2.5));
#34765=CARTESIAN_POINT('Origin',(0.,0.,-2.5));
#34766=CARTESIAN_POINT('Origin',(0.,0.,2.5));
#34767=CARTESIAN_POINT('',(8.,9.79717439317883E-16,2.25));
#34768=CARTESIAN_POINT('',(-8.,-9.79717439317883E-16,2.25));
#34769=CARTESIAN_POINT('Origin',(0.,0.,2.25));
#34770=CARTESIAN_POINT('Origin',(0.,0.,2.25));
#34771=CARTESIAN_POINT('',(-8.,-9.79717439317883E-16,2.5));
#34772=CARTESIAN_POINT('Origin',(0.,0.,2.25));
#34773=CARTESIAN_POINT('',(7.75,-9.49101269339199E-16,2.5));
#34774=CARTESIAN_POINT('',(8.,-9.79717439317883E-16,2.25));
#34775=CARTESIAN_POINT('Origin',(0.,0.,2.5));
#34776=CARTESIAN_POINT('Origin',(0.,7.75,-2.5));
#34777=CARTESIAN_POINT('Origin',(0.,7.75,2.5));
#34778=CARTESIAN_POINT('Origin',(0.,0.,2.5));
#34779=CARTESIAN_POINT('',(-4.76648351648352,-5.83725878165016E-16,2.5));
#34780=CARTESIAN_POINT('Origin',(0.,0.,2.5));
#34781=CARTESIAN_POINT('',(-4.76648351648352,-5.83725878165016E-16,1.11111111111111));
#34782=CARTESIAN_POINT('',(-4.76648351648352,-5.83725878165016E-16,2.5));
#34783=CARTESIAN_POINT('Origin',(0.,0.,1.11111111111111));
#34784=CARTESIAN_POINT('Origin',(0.,0.,-7.04171909509728E-16));
#34785=CARTESIAN_POINT('',(-4.03824256096085,-4.94542082646132E-16,-4.33680868994202E-16));
#34786=CARTESIAN_POINT('Origin',(-5.25,-6.42939569552361E-16,-7.04171909509728E-16));
#34787=CARTESIAN_POINT('Origin',(0.,0.,-4.33680868994202E-16));
#34788=CARTESIAN_POINT('Origin',(0.,0.,2.5));
#34789=CARTESIAN_POINT('',(-3.26912128048043,-4.00351891216485E-16,-2.22044604925031E-15));
#34790=CARTESIAN_POINT('Origin',(0.,0.,-2.16840434497101E-15));
#34791=CARTESIAN_POINT('',(-3.26912128048043,-4.00351891216485E-16,1.75131888199846));
#34792=CARTESIAN_POINT('',(-3.26912128048043,-4.00351891216486E-16,2.5));
#34793=CARTESIAN_POINT('Origin',(0.,0.,1.75131888199846));
#34794=CARTESIAN_POINT('Origin',(0.,0.,2.5));
#34795=CARTESIAN_POINT('',(-4.01780239848197,-4.92038884690751E-16,2.5));
#34796=CARTESIAN_POINT('',(-4.01780239848197,-4.9203888469075E-16,2.5));
#34797=CARTESIAN_POINT('Origin',(0.,0.,2.5));
#34798=CARTESIAN_POINT('Origin',(0.,4.76648351648352,2.5));
#34799=CARTESIAN_POINT('Origin',(0.,3.26912128048043,-1.32068860796267E-15));
#34800=CARTESIAN_POINT('Origin',(0.,0.,2.5));
#34801=CARTESIAN_POINT('',(-2.5,-3.06161699786838E-16,1.73087871951958));
#34802=CARTESIAN_POINT('Origin',(0.,0.,1.73087871951958));
#34803=CARTESIAN_POINT('',(-3.26912128048043,-4.00351891216485E-16,2.5));
#34804=CARTESIAN_POINT('',(-3.26912128048043,-4.00351891216486E-16,2.5));
#34805=CARTESIAN_POINT('Origin',(0.,0.,2.5));
#34806=CARTESIAN_POINT('Origin',(0.,0.,2.5));
#34807=CARTESIAN_POINT('',(2.5,3.2146978477618E-16,-2.25));
#34808=CARTESIAN_POINT('',(-2.5,-3.06161699786838E-16,-2.25));
#34809=CARTESIAN_POINT('Origin',(0.,0.,-2.25));
#34810=CARTESIAN_POINT('Origin',(0.,0.,-2.25));
#34811=CARTESIAN_POINT('',(-2.5,-3.06161699786838E-16,2.5));
#34812=CARTESIAN_POINT('Origin',(0.,0.,-2.25));
#34813=CARTESIAN_POINT('',(2.75,-3.36777869765522E-16,-2.5));
#34814=CARTESIAN_POINT('',(2.5,-3.06161699786838E-16,-2.25));
#34815=CARTESIAN_POINT('Origin',(0.,0.,-2.5));
#34816=CARTESIAN_POINT('Origin',(0.,0.,2.5));
#34817=CARTESIAN_POINT('',(-4.76648351648352,-5.83725878165016E-16,-1.11111111111111));
#34818=CARTESIAN_POINT('Origin',(0.,0.,-1.11111111111111));
#34819=CARTESIAN_POINT('',(-4.76648351648352,-5.83725878165016E-16,-2.5));
#34820=CARTESIAN_POINT('',(-4.76648351648352,-5.83725878165016E-16,2.5));
#34821=CARTESIAN_POINT('Origin',(0.,0.,-2.5));
#34822=CARTESIAN_POINT('Origin',(0.,0.,-7.04171909509728E-16));
#34823=CARTESIAN_POINT('',(-4.03824256096085,-4.94542082646132E-16,-8.67361737988404E-16));
#34824=CARTESIAN_POINT('Origin',(0.,0.,-8.67361737988404E-16));
#34825=CARTESIAN_POINT('Origin',(-5.25,-6.42939569552361E-16,-7.04171909509728E-16));
#34826=CARTESIAN_POINT('Origin',(0.,0.,2.5));
#34827=CARTESIAN_POINT('',(-3.26912128048043,-4.00351891216485E-16,1.75131888199846));
#34828=CARTESIAN_POINT('Origin',(0.,0.,1.75131888199846));
#34829=CARTESIAN_POINT('',(-3.26912128048043,-4.00351891216485E-16,-2.22044604925031E-15));
#34830=CARTESIAN_POINT('',(-3.26912128048043,-4.00351891216486E-16,2.5));
#34831=CARTESIAN_POINT('Origin',(0.,0.,-2.16840434497101E-15));
#34832=CARTESIAN_POINT('Origin',(0.,0.,1.75131888199846));
#34833=CARTESIAN_POINT('',(-4.01780239848197,-4.92038884690751E-16,2.5));
#34834=CARTESIAN_POINT('Origin',(0.,0.,2.5));
#34835=CARTESIAN_POINT('',(-3.26912128048043,-4.00351891216486E-16,1.75131888199846));
#34836=CARTESIAN_POINT('Origin',(0.,4.01780239848197,2.5));
#34837=CARTESIAN_POINT('Origin',(0.,3.26912128048043,-1.51358163738168E-15));
#34838=CARTESIAN_POINT('Origin',(0.,2.75,-2.5));
#34839=CARTESIAN_POINT('Origin',(0.,5.25,-7.04171909509728E-16));
#34840=CARTESIAN_POINT('',(-1.21175743903915,5.25,-7.04171909509728E-16));
#34841=CARTESIAN_POINT('',(1.21175743903915,5.25,-7.04171909509728E-16));
#34842=CARTESIAN_POINT('Origin',(0.,5.25,-7.04171909509728E-16));
#34843=CARTESIAN_POINT('Origin',(3.08587257453549,4.24733922046847,-7.04171909509728E-16));
#34844=CARTESIAN_POINT('',(2.10554021329255,4.95959237249138,-7.04171909509728E-16));
#34845=CARTESIAN_POINT('',(4.06620493577843,3.53508606844556,-7.04171909509728E-16));
#34846=CARTESIAN_POINT('Origin',(3.08587257453549,4.24733922046847,-7.04171909509728E-16));
#34847=CARTESIAN_POINT('Origin',(4.99304671054956,1.62233922046846,-7.04171909509728E-16));
#34848=CARTESIAN_POINT('',(4.6185930688262,2.77478902903577,-7.04171909509728E-16));
#34849=CARTESIAN_POINT('',(5.36750035227292,0.469889411901148,-7.04171909509728E-16));
#34850=CARTESIAN_POINT('Origin',(4.99304671054956,1.62233922046846,-7.04171909509728E-16));
#34851=CARTESIAN_POINT('Origin',(4.99304671054955,-1.6223392204685,-7.04171909509728E-16));
#34852=CARTESIAN_POINT('',(5.36750035227292,-0.469889411901191,-7.04171909509728E-16));
#34853=CARTESIAN_POINT('',(4.61859306882618,-2.77478902903581,-7.04171909509728E-16));
#34854=CARTESIAN_POINT('Origin',(4.99304671054955,-1.6223392204685,-7.04171909509728E-16));
#34855=CARTESIAN_POINT('Origin',(3.08587257453546,-4.24733922046849,-7.04171909509728E-16));
#34856=CARTESIAN_POINT('',(4.0662049357784,-3.53508606844559,-7.04171909509728E-16));
#34857=CARTESIAN_POINT('',(2.10554021329252,-4.95959237249139,-7.04171909509728E-16));
#34858=CARTESIAN_POINT('Origin',(3.08587257453546,-4.24733922046849,-7.04171909509728E-16));
#34859=CARTESIAN_POINT('Origin',(-3.66605540578529E-14,-5.25,-7.04171909509728E-16));
#34860=CARTESIAN_POINT('',(1.21175743903911,-5.25000000000001,-7.04171909509728E-16));
#34861=CARTESIAN_POINT('',(-1.21175743903919,-5.24999999999999,-7.04171909509728E-16));
#34862=CARTESIAN_POINT('Origin',(-3.66605540578529E-14,-5.25,-7.04171909509728E-16));
#34863=CARTESIAN_POINT('Origin',(-3.08587257453552,-4.24733922046845,-7.04171909509728E-16));
#34864=CARTESIAN_POINT('',(-2.10554021329259,-4.95959237249137,-7.04171909509728E-16));
#34865=CARTESIAN_POINT('',(-4.06620493577845,-3.53508606844553,-7.04171909509728E-16));
#34866=CARTESIAN_POINT('Origin',(-3.08587257453552,-4.24733922046845,-7.04171909509728E-16));
#34867=CARTESIAN_POINT('Origin',(-4.99304671054957,-1.62233922046843,-7.04171909509728E-16));
#34868=CARTESIAN_POINT('',(-4.61859306882622,-2.77478902903574,-7.04171909509728E-16));
#34869=CARTESIAN_POINT('',(-5.36750035227292,-0.469889411901115,-7.04171909509728E-16));
#34870=CARTESIAN_POINT('Origin',(-4.99304671054957,-1.62233922046843,-7.04171909509728E-16));
#34871=CARTESIAN_POINT('Origin',(-4.99304671054954,1.62233922046853,-7.04171909509728E-16));
#34872=CARTESIAN_POINT('',(-5.36750035227291,0.469889411901223,-7.04171909509728E-16));
#34873=CARTESIAN_POINT('',(-4.61859306882617,2.77478902903584,-7.04171909509728E-16));
#34874=CARTESIAN_POINT('Origin',(-4.99304671054954,1.62233922046853,-7.04171909509728E-16));
#34875=CARTESIAN_POINT('Origin',(-3.08587257453543,4.24733922046851,-7.04171909509728E-16));
#34876=CARTESIAN_POINT('',(-4.06620493577838,3.53508606844562,-7.04171909509728E-16));
#34877=CARTESIAN_POINT('',(-2.10554021329248,4.95959237249141,-7.04171909509728E-16));
#34878=CARTESIAN_POINT('Origin',(-3.08587257453543,4.24733922046851,-7.04171909509728E-16));
#36435=UNCERTAINTY_MEASURE_WITH_UNIT(LENGTH_MEASURE(0.01),#36461,
'DISTANCE_ACCURACY_VALUE',
'Maximum model space distance between geometric entities at asserted c
onnectivities');
#36444=UNCERTAINTY_MEASURE_WITH_UNIT(LENGTH_MEASURE(0.01),#36461,
'DISTANCE_ACCURACY_VALUE',
'Maximum model space distance between geometric entities at asserted c
onnectivities');
#36451=(
GEOMETRIC_REPRESENTATION_CONTEXT(3)
GLOBAL_UNCERTAINTY_ASSIGNED_CONTEXT((#36435))
GLOBAL_UNIT_ASSIGNED_CONTEXT((#36461,#36463,#36464))
REPRESENTATION_CONTEXT('','3D')
);
#36460=(
GEOMETRIC_REPRESENTATION_CONTEXT(3)
GLOBAL_UNCERTAINTY_ASSIGNED_CONTEXT((#36444))
GLOBAL_UNIT_ASSIGNED_CONTEXT((#36461,#36463,#36464))
REPRESENTATION_CONTEXT('','3D')
);
#36461=(
LENGTH_UNIT()
NAMED_UNIT(*)
SI_UNIT(.MILLI.,.METRE.)
);
#36463=(
NAMED_UNIT(*)
PLANE_ANGLE_UNIT()
SI_UNIT($,.RADIAN.)
);
#36464=(
NAMED_UNIT(*)
SI_UNIT($,.STERADIAN.)
SOLID_ANGLE_UNIT()
);
#36471=SHAPE_DEFINITION_REPRESENTATION(#36486,#36522);
#36486=PRODUCT_DEFINITION_SHAPE('',$,#36538);
#36522=SHAPE_REPRESENTATION('',(#11930),#36451);
#36531=PRODUCT_DEFINITION_CONTEXT('part definition',#36578,'design');
#36538=PRODUCT_DEFINITION(
'5908K51_Highly Corrosion-Resistant 316 Stainless Steel Ball Bearing',
'5908K51_Highly Corrosion-Resistant 316 Stainless Steel Ball Bearing',#36553,
#36531);
#36553=PRODUCT_DEFINITION_FORMATION('',$,#36586);
#36578=APPLICATION_CONTEXT(
'Core Data for Automotive Mechanical Design Process');
#36579=PRODUCT_CONTEXT('part definition',#36578,'mechanical');
#36586=PRODUCT(
'5908K51_Highly Corrosion-Resistant 316 Stainless Steel Ball Bearing',
'5908K51_Highly Corrosion-Resistant 316 Stainless Steel Ball Bearing',$,
(#36579));
#36596=PRESENTATION_STYLE_ASSIGNMENT((#36601));
#36601=SURFACE_STYLE_USAGE(.BOTH.,#36606);
#36606=SURFACE_SIDE_STYLE('',(#36611));
#36611=SURFACE_STYLE_FILL_AREA(#36616);
#36616=FILL_AREA_STYLE('Opaque(160,160,160)',(#36621));
#36621=FILL_AREA_STYLE_COLOUR('Opaque(160,160,160)',#36626);
#36626=COLOUR_RGB('Opaque(160,160,160)', 0.09019608, 0.27058824, 0.51372549);
ENDSEC;
END-ISO-10303-21;
